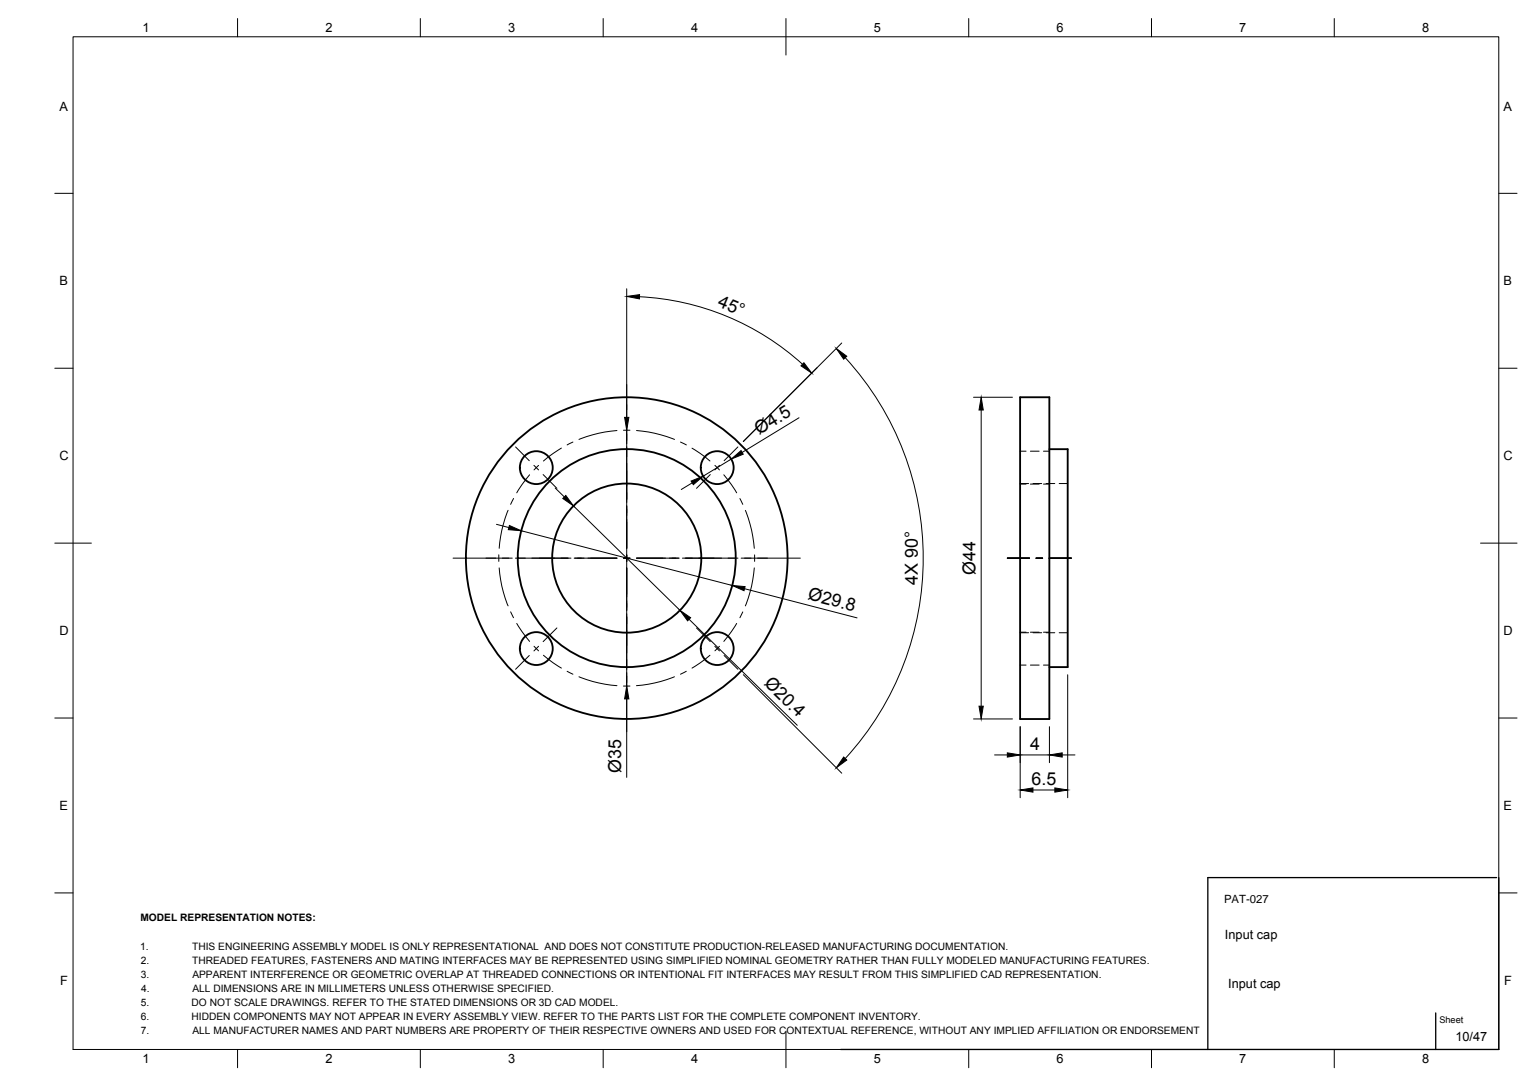
ISO-10303-21;
HEADER;
/* Generated by software containing ST-Developer
 * from STEP Tools, Inc. (www.steptools.com) 
 */

FILE_DESCRIPTION(
/* description */ ('Crank-driven oscillating fan base (mechanism only)'),

/* implementation_level */ '2;1');

FILE_NAME(
/* name */ 'Input cap.step',
/* time_stamp */ '2026-10-28T03:25:00-07:00',
/* author */ (''),
/* organization */ (''),
/* preprocessor_version */ 'ST-DEVELOPER v20.2',
/* originating_system */ 'Autodesk Translation Framework v15.17.0.0',
/* authorisation */ '');

FILE_SCHEMA (('AUTOMOTIVE_DESIGN { 1 0 10303 214 3 1 1 }'));
ENDSEC;

DATA;
#10=MECHANICAL_DESIGN_GEOMETRIC_PRESENTATION_REPRESENTATION('',(#442),#11916);
#362=SHAPE_REPRESENTATION_RELATIONSHIP('SRR','None',#12086,#402);
#402=ADVANCED_BREP_SHAPE_REPRESENTATION('',(#490),#11877);
#442=STYLED_ITEM('',(#12368),#490);
#490=MANIFOLD_SOLID_BREP('Body1',#6072);
#566=FACE_BOUND('',#1362,.T.);
#567=FACE_BOUND('',#1366,.T.);
#568=FACE_BOUND('',#1367,.T.);
#569=FACE_BOUND('',#1368,.T.);
#570=FACE_BOUND('',#1369,.T.);
#571=FACE_BOUND('',#1370,.T.);
#572=FACE_BOUND('',#1372,.T.);
#573=FACE_BOUND('',#1373,.T.);
#574=FACE_BOUND('',#1374,.T.);
#575=FACE_BOUND('',#1375,.T.);
#576=FACE_BOUND('',#1376,.T.);
#724=PLANE('',#6701);
#725=PLANE('',#6708);
#726=PLANE('',#6709);
#945=FACE_OUTER_BOUND('',#1356,.T.);
#946=FACE_OUTER_BOUND('',#1357,.T.);
#947=FACE_OUTER_BOUND('',#1358,.T.);
#948=FACE_OUTER_BOUND('',#1359,.T.);
#949=FACE_OUTER_BOUND('',#1360,.T.);
#950=FACE_OUTER_BOUND('',#1361,.T.);
#951=FACE_OUTER_BOUND('',#1363,.T.);
#952=FACE_OUTER_BOUND('',#1364,.T.);
#953=FACE_OUTER_BOUND('',#1365,.T.);
#954=FACE_OUTER_BOUND('',#1371,.T.);
#1356=EDGE_LOOP('',(#4330,#4331,#4332,#4333));
#1357=EDGE_LOOP('',(#4334,#4335,#4336,#4337));
#1358=EDGE_LOOP('',(#4338,#4339,#4340,#4341));
#1359=EDGE_LOOP('',(#4342,#4343,#4344,#4345));
#1360=EDGE_LOOP('',(#4346,#4347,#4348,#4349));
#1361=EDGE_LOOP('',(#4350));
#1362=EDGE_LOOP('',(#4351));
#1363=EDGE_LOOP('',(#4352,#4353,#4354,#4355));
#1364=EDGE_LOOP('',(#4356,#4357,#4358,#4359));
#1365=EDGE_LOOP('',(#4360));
#1366=EDGE_LOOP('',(#4361));
#1367=EDGE_LOOP('',(#4362));
#1368=EDGE_LOOP('',(#4363));
#1369=EDGE_LOOP('',(#4364));
#1370=EDGE_LOOP('',(#4365));
#1371=EDGE_LOOP('',(#4366));
#1372=EDGE_LOOP('',(#4367));
#1373=EDGE_LOOP('',(#4368));
#1374=EDGE_LOOP('',(#4369));
#1375=EDGE_LOOP('',(#4370));
#1376=EDGE_LOOP('',(#4371));
#1865=LINE('',#9806,#2198);
#1866=LINE('',#9812,#2199);
#1867=LINE('',#9818,#2200);
#1868=LINE('',#9824,#2201);
#1869=LINE('',#9830,#2202);
#1870=LINE('',#9838,#2203);
#1871=LINE('',#9843,#2204);
#2198=VECTOR('',#7736,0.225);
#2199=VECTOR('',#7743,0.225);
#2200=VECTOR('',#7750,0.225);
#2201=VECTOR('',#7757,0.225);
#2202=VECTOR('',#7764,1.49);
#2203=VECTOR('',#7775,1.02);
#2204=VECTOR('',#7780,2.2);
#2524=CIRCLE('',#6687,0.225);
#2525=CIRCLE('',#6688,0.225);
#2526=CIRCLE('',#6690,0.225);
#2527=CIRCLE('',#6691,0.225);
#2528=CIRCLE('',#6693,0.225);
#2529=CIRCLE('',#6694,0.225);
#2530=CIRCLE('',#6696,0.225);
#2531=CIRCLE('',#6697,0.225);
#2532=CIRCLE('',#6699,1.49);
#2533=CIRCLE('',#6700,1.49);
#2534=CIRCLE('',#6702,1.02);
#2535=CIRCLE('',#6704,1.02);
#2536=CIRCLE('',#6706,2.2);
#2537=CIRCLE('',#6707,2.2);
#2917=VERTEX_POINT('',#9803);
#2918=VERTEX_POINT('',#9805);
#2919=VERTEX_POINT('',#9809);
#2920=VERTEX_POINT('',#9811);
#2921=VERTEX_POINT('',#9815);
#2922=VERTEX_POINT('',#9817);
#2923=VERTEX_POINT('',#9821);
#2924=VERTEX_POINT('',#9823);
#2925=VERTEX_POINT('',#9827);
#2926=VERTEX_POINT('',#9829);
#2927=VERTEX_POINT('',#9833);
#2928=VERTEX_POINT('',#9836);
#2929=VERTEX_POINT('',#9840);
#2930=VERTEX_POINT('',#9842);
#3460=EDGE_CURVE('',#2917,#2917,#2524,.T.);
#3461=EDGE_CURVE('',#2917,#2918,#1865,.T.);
#3462=EDGE_CURVE('',#2918,#2918,#2525,.T.);
#3463=EDGE_CURVE('',#2919,#2919,#2526,.T.);
#3464=EDGE_CURVE('',#2919,#2920,#1866,.T.);
#3465=EDGE_CURVE('',#2920,#2920,#2527,.T.);
#3466=EDGE_CURVE('',#2921,#2921,#2528,.T.);
#3467=EDGE_CURVE('',#2921,#2922,#1867,.T.);
#3468=EDGE_CURVE('',#2922,#2922,#2529,.T.);
#3469=EDGE_CURVE('',#2923,#2923,#2530,.T.);
#3470=EDGE_CURVE('',#2923,#2924,#1868,.T.);
#3471=EDGE_CURVE('',#2924,#2924,#2531,.T.);
#3472=EDGE_CURVE('',#2925,#2925,#2532,.T.);
#3473=EDGE_CURVE('',#2925,#2926,#1869,.T.);
#3474=EDGE_CURVE('',#2926,#2926,#2533,.T.);
#3475=EDGE_CURVE('',#2927,#2927,#2534,.T.);
#3476=EDGE_CURVE('',#2928,#2928,#2535,.T.);
#3477=EDGE_CURVE('',#2928,#2927,#1870,.T.);
#3478=EDGE_CURVE('',#2929,#2929,#2536,.T.);
#3479=EDGE_CURVE('',#2929,#2930,#1871,.T.);
#3480=EDGE_CURVE('',#2930,#2930,#2537,.T.);
#4330=ORIENTED_EDGE('',*,*,#3460,.F.);
#4331=ORIENTED_EDGE('',*,*,#3461,.T.);
#4332=ORIENTED_EDGE('',*,*,#3462,.F.);
#4333=ORIENTED_EDGE('',*,*,#3461,.F.);
#4334=ORIENTED_EDGE('',*,*,#3463,.F.);
#4335=ORIENTED_EDGE('',*,*,#3464,.T.);
#4336=ORIENTED_EDGE('',*,*,#3465,.F.);
#4337=ORIENTED_EDGE('',*,*,#3464,.F.);
#4338=ORIENTED_EDGE('',*,*,#3466,.F.);
#4339=ORIENTED_EDGE('',*,*,#3467,.T.);
#4340=ORIENTED_EDGE('',*,*,#3468,.F.);
#4341=ORIENTED_EDGE('',*,*,#3467,.F.);
#4342=ORIENTED_EDGE('',*,*,#3469,.F.);
#4343=ORIENTED_EDGE('',*,*,#3470,.T.);
#4344=ORIENTED_EDGE('',*,*,#3471,.F.);
#4345=ORIENTED_EDGE('',*,*,#3470,.F.);
#4346=ORIENTED_EDGE('',*,*,#3472,.F.);
#4347=ORIENTED_EDGE('',*,*,#3473,.T.);
#4348=ORIENTED_EDGE('',*,*,#3474,.T.);
#4349=ORIENTED_EDGE('',*,*,#3473,.F.);
#4350=ORIENTED_EDGE('',*,*,#3474,.F.);
#4351=ORIENTED_EDGE('',*,*,#3475,.F.);
#4352=ORIENTED_EDGE('',*,*,#3476,.F.);
#4353=ORIENTED_EDGE('',*,*,#3477,.T.);
#4354=ORIENTED_EDGE('',*,*,#3475,.T.);
#4355=ORIENTED_EDGE('',*,*,#3477,.F.);
#4356=ORIENTED_EDGE('',*,*,#3478,.F.);
#4357=ORIENTED_EDGE('',*,*,#3479,.T.);
#4358=ORIENTED_EDGE('',*,*,#3480,.T.);
#4359=ORIENTED_EDGE('',*,*,#3479,.F.);
#4360=ORIENTED_EDGE('',*,*,#3478,.T.);
#4361=ORIENTED_EDGE('',*,*,#3476,.T.);
#4362=ORIENTED_EDGE('',*,*,#3471,.T.);
#4363=ORIENTED_EDGE('',*,*,#3468,.T.);
#4364=ORIENTED_EDGE('',*,*,#3465,.T.);
#4365=ORIENTED_EDGE('',*,*,#3462,.T.);
#4366=ORIENTED_EDGE('',*,*,#3480,.F.);
#4367=ORIENTED_EDGE('',*,*,#3472,.T.);
#4368=ORIENTED_EDGE('',*,*,#3469,.T.);
#4369=ORIENTED_EDGE('',*,*,#3466,.T.);
#4370=ORIENTED_EDGE('',*,*,#3463,.T.);
#4371=ORIENTED_EDGE('',*,*,#3460,.T.);
#5573=CYLINDRICAL_SURFACE('',#6686,0.225);
#5574=CYLINDRICAL_SURFACE('',#6689,0.225);
#5575=CYLINDRICAL_SURFACE('',#6692,0.225);
#5576=CYLINDRICAL_SURFACE('',#6695,0.225);
#5577=CYLINDRICAL_SURFACE('',#6698,1.49);
#5578=CYLINDRICAL_SURFACE('',#6703,1.02);
#5579=CYLINDRICAL_SURFACE('',#6705,2.2);
#5751=ADVANCED_FACE('',(#945),#5573,.F.);
#5752=ADVANCED_FACE('',(#946),#5574,.F.);
#5753=ADVANCED_FACE('',(#947),#5575,.F.);
#5754=ADVANCED_FACE('',(#948),#5576,.F.);
#5755=ADVANCED_FACE('',(#949),#5577,.T.);
#5756=ADVANCED_FACE('',(#950,#566),#724,.F.);
#5757=ADVANCED_FACE('',(#951),#5578,.F.);
#5758=ADVANCED_FACE('',(#952),#5579,.T.);
#5759=ADVANCED_FACE('',(#953,#567,#568,#569,#570,#571),#725,.T.);
#5760=ADVANCED_FACE('',(#954,#572,#573,#574,#575,#576),#726,.F.);
#6072=CLOSED_SHELL('',(#5751,#5752,#5753,#5754,#5755,#5756,#5757,#5758,
#5759,#5760));
#6685=AXIS2_PLACEMENT_3D('',#9801,#7730,#7731);
#6686=AXIS2_PLACEMENT_3D('',#9802,#7732,#7733);
#6687=AXIS2_PLACEMENT_3D('',#9804,#7734,#7735);
#6688=AXIS2_PLACEMENT_3D('',#9807,#7737,#7738);
#6689=AXIS2_PLACEMENT_3D('',#9808,#7739,#7740);
#6690=AXIS2_PLACEMENT_3D('',#9810,#7741,#7742);
#6691=AXIS2_PLACEMENT_3D('',#9813,#7744,#7745);
#6692=AXIS2_PLACEMENT_3D('',#9814,#7746,#7747);
#6693=AXIS2_PLACEMENT_3D('',#9816,#7748,#7749);
#6694=AXIS2_PLACEMENT_3D('',#9819,#7751,#7752);
#6695=AXIS2_PLACEMENT_3D('',#9820,#7753,#7754);
#6696=AXIS2_PLACEMENT_3D('',#9822,#7755,#7756);
#6697=AXIS2_PLACEMENT_3D('',#9825,#7758,#7759);
#6698=AXIS2_PLACEMENT_3D('',#9826,#7760,#7761);
#6699=AXIS2_PLACEMENT_3D('',#9828,#7762,#7763);
#6700=AXIS2_PLACEMENT_3D('',#9831,#7765,#7766);
#6701=AXIS2_PLACEMENT_3D('',#9832,#7767,#7768);
#6702=AXIS2_PLACEMENT_3D('',#9834,#7769,#7770);
#6703=AXIS2_PLACEMENT_3D('',#9835,#7771,#7772);
#6704=AXIS2_PLACEMENT_3D('',#9837,#7773,#7774);
#6705=AXIS2_PLACEMENT_3D('',#9839,#7776,#7777);
#6706=AXIS2_PLACEMENT_3D('',#9841,#7778,#7779);
#6707=AXIS2_PLACEMENT_3D('',#9844,#7781,#7782);
#6708=AXIS2_PLACEMENT_3D('',#9845,#7783,#7784);
#6709=AXIS2_PLACEMENT_3D('',#9846,#7785,#7786);
#7730=DIRECTION('axis',(0.,0.,1.));
#7731=DIRECTION('refdir',(1.,0.,0.));
#7732=DIRECTION('center_axis',(0.,0.,1.));
#7733=DIRECTION('ref_axis',(1.,0.,0.));
#7734=DIRECTION('center_axis',(0.,0.,1.));
#7735=DIRECTION('ref_axis',(1.,0.,0.));
#7736=DIRECTION('',(0.,0.,1.));
#7737=DIRECTION('center_axis',(0.,0.,-1.));
#7738=DIRECTION('ref_axis',(1.,0.,0.));
#7739=DIRECTION('center_axis',(0.,0.,1.));
#7740=DIRECTION('ref_axis',(1.,0.,0.));
#7741=DIRECTION('center_axis',(0.,0.,1.));
#7742=DIRECTION('ref_axis',(1.,0.,0.));
#7743=DIRECTION('',(0.,0.,1.));
#7744=DIRECTION('center_axis',(0.,0.,-1.));
#7745=DIRECTION('ref_axis',(1.,0.,0.));
#7746=DIRECTION('center_axis',(0.,0.,1.));
#7747=DIRECTION('ref_axis',(1.,0.,0.));
#7748=DIRECTION('center_axis',(0.,0.,1.));
#7749=DIRECTION('ref_axis',(1.,0.,0.));
#7750=DIRECTION('',(0.,0.,1.));
#7751=DIRECTION('center_axis',(0.,0.,-1.));
#7752=DIRECTION('ref_axis',(1.,0.,0.));
#7753=DIRECTION('center_axis',(0.,0.,1.));
#7754=DIRECTION('ref_axis',(1.,0.,0.));
#7755=DIRECTION('center_axis',(0.,0.,1.));
#7756=DIRECTION('ref_axis',(1.,0.,0.));
#7757=DIRECTION('',(0.,0.,1.));
#7758=DIRECTION('center_axis',(0.,0.,-1.));
#7759=DIRECTION('ref_axis',(1.,0.,0.));
#7760=DIRECTION('center_axis',(0.,0.,1.));
#7761=DIRECTION('ref_axis',(1.,0.,0.));
#7762=DIRECTION('center_axis',(0.,0.,1.));
#7763=DIRECTION('ref_axis',(1.,0.,0.));
#7764=DIRECTION('',(0.,0.,-1.));
#7765=DIRECTION('center_axis',(0.,0.,1.));
#7766=DIRECTION('ref_axis',(1.,0.,0.));
#7767=DIRECTION('center_axis',(0.,0.,1.));
#7768=DIRECTION('ref_axis',(1.,0.,0.));
#7769=DIRECTION('center_axis',(0.,0.,-1.));
#7770=DIRECTION('ref_axis',(1.,0.,0.));
#7771=DIRECTION('center_axis',(0.,0.,1.));
#7772=DIRECTION('ref_axis',(1.,0.,0.));
#7773=DIRECTION('center_axis',(0.,0.,-1.));
#7774=DIRECTION('ref_axis',(1.,0.,0.));
#7775=DIRECTION('',(0.,0.,-1.));
#7776=DIRECTION('center_axis',(0.,0.,1.));
#7777=DIRECTION('ref_axis',(1.,0.,0.));
#7778=DIRECTION('center_axis',(0.,0.,1.));
#7779=DIRECTION('ref_axis',(1.,0.,0.));
#7780=DIRECTION('',(0.,0.,-1.));
#7781=DIRECTION('center_axis',(0.,0.,1.));
#7782=DIRECTION('ref_axis',(1.,0.,0.));
#7783=DIRECTION('center_axis',(0.,0.,1.));
#7784=DIRECTION('ref_axis',(1.,0.,0.));
#7785=DIRECTION('center_axis',(0.,0.,1.));
#7786=DIRECTION('ref_axis',(1.,0.,0.));
#9801=CARTESIAN_POINT('',(0.,0.,0.));
#9802=CARTESIAN_POINT('Origin',(-1.23743686707646,-1.23743686707646,5.1));
#9803=CARTESIAN_POINT('',(-1.46243686707646,-1.23743686707646,5.2));
#9804=CARTESIAN_POINT('Origin',(-1.23743686707646,-1.23743686707646,5.2));
#9805=CARTESIAN_POINT('',(-1.46243686707646,-1.23743686707646,5.6));
#9806=CARTESIAN_POINT('',(-1.46243686707646,-1.23743686707646,5.1));
#9807=CARTESIAN_POINT('Origin',(-1.23743686707646,-1.23743686707646,5.6));
#9808=CARTESIAN_POINT('Origin',(-1.23743686707646,1.23743686707646,5.1));
#9809=CARTESIAN_POINT('',(-1.46243686707646,1.23743686707646,5.2));
#9810=CARTESIAN_POINT('Origin',(-1.23743686707646,1.23743686707646,5.2));
#9811=CARTESIAN_POINT('',(-1.46243686707646,1.23743686707646,5.6));
#9812=CARTESIAN_POINT('',(-1.46243686707646,1.23743686707646,5.1));
#9813=CARTESIAN_POINT('Origin',(-1.23743686707646,1.23743686707646,5.6));
#9814=CARTESIAN_POINT('Origin',(1.23743686707646,1.23743686707646,5.1));
#9815=CARTESIAN_POINT('',(1.01243686707646,1.23743686707646,5.2));
#9816=CARTESIAN_POINT('Origin',(1.23743686707646,1.23743686707646,5.2));
#9817=CARTESIAN_POINT('',(1.01243686707646,1.23743686707646,5.6));
#9818=CARTESIAN_POINT('',(1.01243686707646,1.23743686707646,5.1));
#9819=CARTESIAN_POINT('Origin',(1.23743686707646,1.23743686707646,5.6));
#9820=CARTESIAN_POINT('Origin',(1.23743686707646,-1.23743686707646,5.1));
#9821=CARTESIAN_POINT('',(1.01243686707646,-1.23743686707646,5.2));
#9822=CARTESIAN_POINT('Origin',(1.23743686707646,-1.23743686707646,5.2));
#9823=CARTESIAN_POINT('',(1.01243686707646,-1.23743686707646,5.6));
#9824=CARTESIAN_POINT('',(1.01243686707646,-1.23743686707646,5.1));
#9825=CARTESIAN_POINT('Origin',(1.23743686707646,-1.23743686707646,5.6));
#9826=CARTESIAN_POINT('Origin',(0.,0.,4.95));
#9827=CARTESIAN_POINT('',(-1.49,-1.82472373072956E-16,5.2));
#9828=CARTESIAN_POINT('Origin',(0.,0.,5.2));
#9829=CARTESIAN_POINT('',(-1.49,-1.82472373072956E-16,4.95));
#9830=CARTESIAN_POINT('',(-1.49,-1.82472373072956E-16,4.95));
#9831=CARTESIAN_POINT('Origin',(0.,0.,4.95));
#9832=CARTESIAN_POINT('Origin',(0.,0.,4.95));
#9833=CARTESIAN_POINT('',(-1.02,-1.2491397351303E-16,4.95));
#9834=CARTESIAN_POINT('Origin',(0.,0.,4.95));
#9835=CARTESIAN_POINT('Origin',(0.,0.,5.2));
#9836=CARTESIAN_POINT('',(-1.02,-1.2491397351303E-16,5.6));
#9837=CARTESIAN_POINT('Origin',(0.,0.,5.6));
#9838=CARTESIAN_POINT('',(-1.02,-1.2491397351303E-16,5.2));
#9839=CARTESIAN_POINT('Origin',(0.,0.,5.2));
#9840=CARTESIAN_POINT('',(-2.2,-2.69422295812418E-16,5.6));
#9841=CARTESIAN_POINT('Origin',(0.,0.,5.6));
#9842=CARTESIAN_POINT('',(-2.2,-2.69422295812418E-16,5.2));
#9843=CARTESIAN_POINT('',(-2.2,-2.69422295812418E-16,5.2));
#9844=CARTESIAN_POINT('Origin',(0.,0.,5.2));
#9845=CARTESIAN_POINT('Origin',(0.,0.,5.6));
#9846=CARTESIAN_POINT('Origin',(0.,0.,5.2));
#11830=UNCERTAINTY_MEASURE_WITH_UNIT(LENGTH_MEASURE(0.001),#11917,
'DISTANCE_ACCURACY_VALUE',
'Maximum model space distance between geometric entities at asserted c
onnectivities');
#11869=UNCERTAINTY_MEASURE_WITH_UNIT(LENGTH_MEASURE(0.001),#11917,
'DISTANCE_ACCURACY_VALUE',
'Maximum model space distance between geometric entities at asserted c
onnectivities');
#11877=(
GEOMETRIC_REPRESENTATION_CONTEXT(3)
GLOBAL_UNCERTAINTY_ASSIGNED_CONTEXT((#11830))
GLOBAL_UNIT_ASSIGNED_CONTEXT((#11917,#11919,#11920))
REPRESENTATION_CONTEXT('','3D')
);
#11916=(
GEOMETRIC_REPRESENTATION_CONTEXT(3)
GLOBAL_UNCERTAINTY_ASSIGNED_CONTEXT((#11869))
GLOBAL_UNIT_ASSIGNED_CONTEXT((#11917,#11919,#11920))
REPRESENTATION_CONTEXT('','3D')
);
#11917=(
LENGTH_UNIT()
NAMED_UNIT(*)
SI_UNIT(.CENTI.,.METRE.)
);
#11919=(
NAMED_UNIT(*)
PLANE_ANGLE_UNIT()
SI_UNIT($,.RADIAN.)
);
#11920=(
NAMED_UNIT(*)
SI_UNIT($,.STERADIAN.)
SOLID_ANGLE_UNIT()
);
#11928=SHAPE_DEFINITION_REPRESENTATION(#11974,#12086);
#11974=PRODUCT_DEFINITION_SHAPE('',$,#12133);
#12086=SHAPE_REPRESENTATION('',(#6685),#11877);
#12125=PRODUCT_DEFINITION_CONTEXT('part definition',#12265,'design');
#12133=PRODUCT_DEFINITION('Input cap','Input cap',#12179,#12125);
#12179=PRODUCT_DEFINITION_FORMATION('',$,#12274);
#12265=APPLICATION_CONTEXT(
'Core Data for Automotive Mechanical Design Process');
#12266=PRODUCT_CONTEXT('part definition',#12265,'mechanical');
#12274=PRODUCT('Input cap','Input cap','Input cap',(#12266));
#12362=COLOUR_RGB('Sky Blue',0.24,0.69,0.87);
#12363=FILL_AREA_STYLE_COLOUR('',#12362);
#12364=FILL_AREA_STYLE('',(#12363));
#12365=SURFACE_STYLE_FILL_AREA(#12364);
#12366=SURFACE_SIDE_STYLE('',(#12365));
#12367=SURFACE_STYLE_USAGE(.BOTH.,#12366);
#12368=PRESENTATION_STYLE_ASSIGNMENT((#12367));
ENDSEC;
END-ISO-10303-21;
